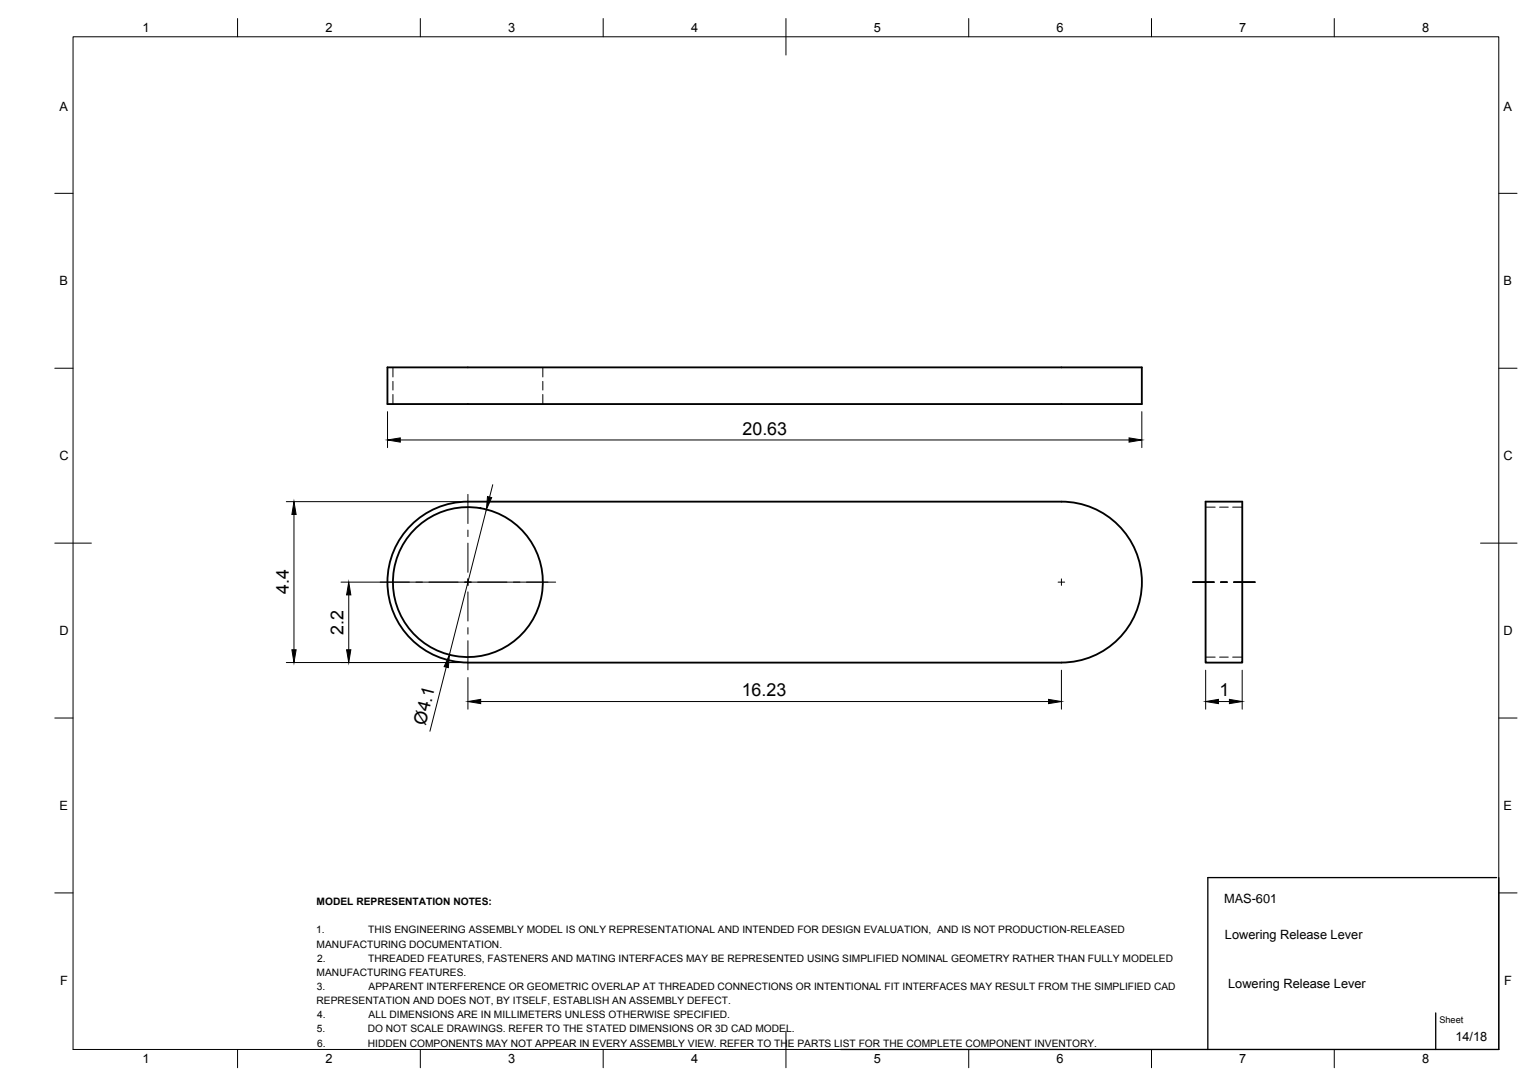
ISO-10303-21;
HEADER;
FILE_DESCRIPTION((''),'2;1');
FILE_NAME('Lowering Release Lever.step','2026-10-06T07:37:42+05:00',(''),(''),'','','');
FILE_SCHEMA (('AUTOMOTIVE_DESIGN { 1 0 10303 214 3 1 1 }'));
ENDSEC;
DATA;
#10=MECHANICAL_DESIGN_GEOMETRIC_PRESENTATION_REPRESENTATION('',(#382),#18757);
#348=SHAPE_REPRESENTATION_RELATIONSHIP('SRR','None',#18866,#365) ;
#365=ADVANCED_BREP_SHAPE_REPRESENTATION('',(#399),#18749) ;
#382=STYLED_ITEM('',(#18960),#399) ;
#399=MANIFOLD_SOLID_BREP('Lowering Release Lever',#9551) ;
#585=CYLINDRICAL_SURFACE('',#10206,2.05) ;
#586=CYLINDRICAL_SURFACE('',#10210,2.2) ;
#587=CYLINDRICAL_SURFACE('',#10214,2.20000000000001) ;
#727=FACE_BOUND('',#1939,.T.) ;
#728=FACE_BOUND('',#1941,.T.) ;
#902=PLANE('',#10209) ;
#903=PLANE('',#10213) ;
#904=PLANE('',#10217) ;
#905=PLANE('',#10218) ;
#1338=FACE_OUTER_BOUND('',#1933,.T.) ;
#1339=FACE_OUTER_BOUND('',#1934,.T.) ;
#1340=FACE_OUTER_BOUND('',#1935,.T.) ;
#1341=FACE_OUTER_BOUND('',#1936,.T.) ;
#1342=FACE_OUTER_BOUND('',#1937,.T.) ;
#1343=FACE_OUTER_BOUND('',#1938,.T.) ;
#1344=FACE_OUTER_BOUND('',#1940,.T.) ;
#1933=EDGE_LOOP('',(#7607,#7608,#7609,#7610)) ;
#1934=EDGE_LOOP('',(#7611,#7612,#7613,#7614)) ;
#1935=EDGE_LOOP('',(#7615,#7616,#7617,#7618)) ;
#1936=EDGE_LOOP('',(#7619,#7620,#7621,#7622)) ;
#1937=EDGE_LOOP('',(#7623,#7624,#7625,#7626)) ;
#1938=EDGE_LOOP('',(#7627,#7628,#7629,#7630)) ;
#1939=EDGE_LOOP('',(#7631)) ;
#1940=EDGE_LOOP('',(#7632,#7633,#7634,#7635)) ;
#1941=EDGE_LOOP('',(#7636)) ;
#2637=LINE('',#15165,#3408) ;
#2638=LINE('',#15170,#3409) ;
#2639=LINE('',#15172,#3410) ;
#2640=LINE('',#15174,#3411) ;
#2641=LINE('',#15175,#3412) ;
#2642=LINE('',#15181,#3413) ;
#2643=LINE('',#15184,#3414) ;
#2644=LINE('',#15186,#3415) ;
#2645=LINE('',#15187,#3416) ;
#3408=VECTOR('',#12041,2.05) ;
#3409=VECTOR('',#12046,10.) ;
#3410=VECTOR('',#12047,10.) ;
#3411=VECTOR('',#12048,10.) ;
#3412=VECTOR('',#12049,10.) ;
#3413=VECTOR('',#12056,10.) ;
#3414=VECTOR('',#12059,10.) ;
#3415=VECTOR('',#12060,10.) ;
#3416=VECTOR('',#12061,10.) ;
#3972=CIRCLE('',#10207,2.05) ;
#3973=CIRCLE('',#10208,2.05) ;
#3974=CIRCLE('',#10211,2.2) ;
#3975=CIRCLE('',#10212,2.2) ;
#3976=CIRCLE('',#10215,2.20000000000001) ;
#3977=CIRCLE('',#10216,2.20000000000001) ;
#4565=VERTEX_POINT('',#15162) ;
#4566=VERTEX_POINT('',#15164) ;
#4567=VERTEX_POINT('',#15168) ;
#4568=VERTEX_POINT('',#15169) ;
#4569=VERTEX_POINT('',#15171) ;
#4570=VERTEX_POINT('',#15173) ;
#4571=VERTEX_POINT('',#15177) ;
#4572=VERTEX_POINT('',#15179) ;
#4573=VERTEX_POINT('',#15183) ;
#4574=VERTEX_POINT('',#15185) ;
#5650=EDGE_CURVE('',#4565,#4565,#3972,.T.) ;
#5651=EDGE_CURVE('',#4565,#4566,#2637,.T.) ;
#5652=EDGE_CURVE('',#4566,#4566,#3973,.T.) ;
#5653=EDGE_CURVE('',#4567,#4568,#2638,.T.) ;
#5654=EDGE_CURVE('',#4568,#4569,#2639,.T.) ;
#5655=EDGE_CURVE('',#4570,#4569,#2640,.T.) ;
#5656=EDGE_CURVE('',#4567,#4570,#2641,.T.) ;
#5657=EDGE_CURVE('',#4571,#4567,#3974,.T.) ;
#5658=EDGE_CURVE('',#4572,#4570,#3975,.T.) ;
#5659=EDGE_CURVE('',#4571,#4572,#2642,.T.) ;
#5660=EDGE_CURVE('',#4573,#4571,#2643,.T.) ;
#5661=EDGE_CURVE('',#4574,#4572,#2644,.T.) ;
#5662=EDGE_CURVE('',#4573,#4574,#2645,.T.) ;
#5663=EDGE_CURVE('',#4568,#4573,#3976,.T.) ;
#5664=EDGE_CURVE('',#4569,#4574,#3977,.T.) ;
#7607=ORIENTED_EDGE('',*,*,#5650,.F.) ;
#7608=ORIENTED_EDGE('',*,*,#5651,.T.) ;
#7609=ORIENTED_EDGE('',*,*,#5652,.T.) ;
#7610=ORIENTED_EDGE('',*,*,#5651,.F.) ;
#7611=ORIENTED_EDGE('',*,*,#5653,.T.) ;
#7612=ORIENTED_EDGE('',*,*,#5654,.T.) ;
#7613=ORIENTED_EDGE('',*,*,#5655,.F.) ;
#7614=ORIENTED_EDGE('',*,*,#5656,.F.) ;
#7615=ORIENTED_EDGE('',*,*,#5657,.T.) ;
#7616=ORIENTED_EDGE('',*,*,#5656,.T.) ;
#7617=ORIENTED_EDGE('',*,*,#5658,.F.) ;
#7618=ORIENTED_EDGE('',*,*,#5659,.F.) ;
#7619=ORIENTED_EDGE('',*,*,#5660,.T.) ;
#7620=ORIENTED_EDGE('',*,*,#5659,.T.) ;
#7621=ORIENTED_EDGE('',*,*,#5661,.F.) ;
#7622=ORIENTED_EDGE('',*,*,#5662,.F.) ;
#7623=ORIENTED_EDGE('',*,*,#5663,.T.) ;
#7624=ORIENTED_EDGE('',*,*,#5662,.T.) ;
#7625=ORIENTED_EDGE('',*,*,#5664,.F.) ;
#7626=ORIENTED_EDGE('',*,*,#5654,.F.) ;
#7627=ORIENTED_EDGE('',*,*,#5664,.T.) ;
#7628=ORIENTED_EDGE('',*,*,#5661,.T.) ;
#7629=ORIENTED_EDGE('',*,*,#5658,.T.) ;
#7630=ORIENTED_EDGE('',*,*,#5655,.T.) ;
#7631=ORIENTED_EDGE('',*,*,#5650,.T.) ;
#7632=ORIENTED_EDGE('',*,*,#5663,.F.) ;
#7633=ORIENTED_EDGE('',*,*,#5653,.F.) ;
#7634=ORIENTED_EDGE('',*,*,#5657,.F.) ;
#7635=ORIENTED_EDGE('',*,*,#5660,.F.) ;
#7636=ORIENTED_EDGE('',*,*,#5652,.F.) ;
#9274=ADVANCED_FACE('',(#1338),#585,.F.) ;
#9275=ADVANCED_FACE('',(#1339),#902,.T.) ;
#9276=ADVANCED_FACE('',(#1340),#586,.T.) ;
#9277=ADVANCED_FACE('',(#1341),#903,.T.) ;
#9278=ADVANCED_FACE('',(#1342),#587,.T.) ;
#9279=ADVANCED_FACE('',(#1343,#727),#904,.T.) ;
#9280=ADVANCED_FACE('',(#1344,#728),#905,.F.) ;
#9551=CLOSED_SHELL('',(#9274,#9275,#9276,#9277,#9278,#9279,#9280)) ;
#10205=AXIS2_PLACEMENT_3D('',#15160,#12035,#12036) ;
#10206=AXIS2_PLACEMENT_3D('',#15161,#12037,#12038) ;
#10207=AXIS2_PLACEMENT_3D('',#15163,#12039,#12040) ;
#10208=AXIS2_PLACEMENT_3D('',#15166,#12042,#12043) ;
#10209=AXIS2_PLACEMENT_3D('',#15167,#12044,#12045) ;
#10210=AXIS2_PLACEMENT_3D('',#15176,#12050,#12051) ;
#10211=AXIS2_PLACEMENT_3D('',#15178,#12052,#12053) ;
#10212=AXIS2_PLACEMENT_3D('',#15180,#12054,#12055) ;
#10213=AXIS2_PLACEMENT_3D('',#15182,#12057,#12058) ;
#10214=AXIS2_PLACEMENT_3D('',#15188,#12062,#12063) ;
#10215=AXIS2_PLACEMENT_3D('',#15189,#12064,#12065) ;
#10216=AXIS2_PLACEMENT_3D('',#15190,#12066,#12067) ;
#10217=AXIS2_PLACEMENT_3D('',#15191,#12068,#12069) ;
#10218=AXIS2_PLACEMENT_3D('',#15192,#12070,#12071) ;
#12035=DIRECTION('axis',(0.,0.,1.)) ;
#12036=DIRECTION('refdir',(1.,0.,0.)) ;
#12037=DIRECTION('center_axis',(0.,1.,0.)) ;
#12038=DIRECTION('ref_axis',(1.,0.,0.)) ;
#12039=DIRECTION('center_axis',(0.,-1.,0.)) ;
#12040=DIRECTION('ref_axis',(1.,0.,0.)) ;
#12041=DIRECTION('',(0.,-1.,0.)) ;
#12042=DIRECTION('center_axis',(0.,-1.,0.)) ;
#12043=DIRECTION('ref_axis',(1.,0.,0.)) ;
#12044=DIRECTION('center_axis',(0.985548890759753,0.,-0.169391215599333)) ;
#12045=DIRECTION('ref_axis',(-0.169391215599333,0.,-0.985548890759753)) ;
#12046=DIRECTION('',(-0.169391215599333,0.,-0.985548890759753)) ;
#12047=DIRECTION('',(0.,1.,0.)) ;
#12048=DIRECTION('',(-0.169391215599333,0.,-0.985548890759753)) ;
#12049=DIRECTION('',(0.,1.,0.)) ;
#12050=DIRECTION('center_axis',(0.,1.,0.)) ;
#12051=DIRECTION('ref_axis',(-0.985548890759752,0.,0.169391215599339)) ;
#12052=DIRECTION('center_axis',(0.,1.,0.)) ;
#12053=DIRECTION('ref_axis',(-0.985548890759752,0.,0.169391215599339)) ;
#12054=DIRECTION('center_axis',(0.,1.,0.)) ;
#12055=DIRECTION('ref_axis',(-0.985548890759752,0.,0.169391215599339)) ;
#12056=DIRECTION('',(0.,1.,0.)) ;
#12057=DIRECTION('center_axis',(-0.985548890759753,0.,0.169391215599333)) ;
#12058=DIRECTION('ref_axis',(0.169391215599333,0.,0.985548890759753)) ;
#12059=DIRECTION('',(0.169391215599333,0.,0.985548890759753)) ;
#12060=DIRECTION('',(0.169391215599333,0.,0.985548890759753)) ;
#12061=DIRECTION('',(0.,1.,0.)) ;
#12062=DIRECTION('center_axis',(0.,1.,0.)) ;
#12063=DIRECTION('ref_axis',(0.985548890759754,0.,-0.16939121559933)) ;
#12064=DIRECTION('center_axis',(0.,1.,0.)) ;
#12065=DIRECTION('ref_axis',(0.985548890759754,0.,-0.16939121559933)) ;
#12066=DIRECTION('center_axis',(0.,1.,0.)) ;
#12067=DIRECTION('ref_axis',(0.985548890759754,0.,-0.16939121559933)) ;
#12068=DIRECTION('center_axis',(0.,1.,0.)) ;
#12069=DIRECTION('ref_axis',(1.,0.,0.)) ;
#12070=DIRECTION('center_axis',(0.,1.,0.)) ;
#12071=DIRECTION('ref_axis',(1.,0.,0.)) ;
#15160=CARTESIAN_POINT('',(0.,0.,0.)) ;
#15161=CARTESIAN_POINT('Origin',(90.25,47.1,160.)) ;
#15162=CARTESIAN_POINT('',(88.2,48.1,160.)) ;
#15163=CARTESIAN_POINT('Origin',(90.25,48.1,160.)) ;
#15164=CARTESIAN_POINT('',(88.2,47.1,160.)) ;
#15165=CARTESIAN_POINT('',(88.2,47.1,160.)) ;
#15166=CARTESIAN_POINT('Origin',(90.25,47.1,160.)) ;
#15167=CARTESIAN_POINT('Origin',(95.1682075596715,47.1,175.627339325681)) ;
#15168=CARTESIAN_POINT('',(95.1682075596715,47.1,175.627339325681)) ;
#15169=CARTESIAN_POINT('',(92.4182075596715,47.1,159.627339325681)) ;
#15170=CARTESIAN_POINT('',(95.1682075596715,47.1,175.627339325681)) ;
#15171=CARTESIAN_POINT('',(92.4182075596715,48.1,159.627339325681)) ;
#15172=CARTESIAN_POINT('',(92.4182075596715,47.1,159.627339325681)) ;
#15173=CARTESIAN_POINT('',(95.1682075596715,48.1,175.627339325681)) ;
#15174=CARTESIAN_POINT('',(95.1682075596715,48.1,175.627339325681)) ;
#15175=CARTESIAN_POINT('',(95.1682075596715,47.1,175.627339325681)) ;
#15176=CARTESIAN_POINT('Origin',(93.,47.1,176.)) ;
#15177=CARTESIAN_POINT('',(90.8317924403285,47.1,176.372660674319)) ;
#15178=CARTESIAN_POINT('Origin',(93.,47.1,176.)) ;
#15179=CARTESIAN_POINT('',(90.8317924403285,48.1,176.372660674319)) ;
#15180=CARTESIAN_POINT('Origin',(93.,48.1,176.)) ;
#15181=CARTESIAN_POINT('',(90.8317924403285,47.1,176.372660674319)) ;
#15182=CARTESIAN_POINT('Origin',(88.0817924403285,47.1,160.372660674319)) ;
#15183=CARTESIAN_POINT('',(88.0817924403285,47.1,160.372660674319)) ;
#15184=CARTESIAN_POINT('',(88.0817924403285,47.1,160.372660674319)) ;
#15185=CARTESIAN_POINT('',(88.0817924403285,48.1,160.372660674319)) ;
#15186=CARTESIAN_POINT('',(88.0817924403285,48.1,160.372660674319)) ;
#15187=CARTESIAN_POINT('',(88.0817924403285,47.1,160.372660674319)) ;
#15188=CARTESIAN_POINT('Origin',(90.25,47.1,160.)) ;
#15189=CARTESIAN_POINT('Origin',(90.25,47.1,160.)) ;
#15190=CARTESIAN_POINT('Origin',(90.25,48.1,160.)) ;
#15191=CARTESIAN_POINT('Origin',(91.625,48.1,168.)) ;
#15192=CARTESIAN_POINT('Origin',(91.625,47.1,168.)) ;
#18730=UNCERTAINTY_MEASURE_WITH_UNIT(LENGTH_MEASURE(0.01),#18758,
'DISTANCE_ACCURACY_VALUE',
'Maximum model space distance between geometric entities at asserted c
onnectivities') ;
#18738=UNCERTAINTY_MEASURE_WITH_UNIT(LENGTH_MEASURE(0.01),#18758,
'DISTANCE_ACCURACY_VALUE',
'Maximum model space distance between geometric entities at asserted c
onnectivities') ;
#18749=(
GEOMETRIC_REPRESENTATION_CONTEXT(3)
GLOBAL_UNCERTAINTY_ASSIGNED_CONTEXT((#18730))
GLOBAL_UNIT_ASSIGNED_CONTEXT((#18758,#18760,#18761))
REPRESENTATION_CONTEXT('','3D')
) ;
#18757=(
GEOMETRIC_REPRESENTATION_CONTEXT(3)
GLOBAL_UNCERTAINTY_ASSIGNED_CONTEXT((#18738))
GLOBAL_UNIT_ASSIGNED_CONTEXT((#18758,#18760,#18761))
REPRESENTATION_CONTEXT('','3D')
) ;
#18758=(
LENGTH_UNIT()
NAMED_UNIT(*)
SI_UNIT(.MILLI.,.METRE.)
) ;
#18760=(
NAMED_UNIT(*)
PLANE_ANGLE_UNIT()
SI_UNIT($,.RADIAN.)
) ;
#18761=(
NAMED_UNIT(*)
SI_UNIT($,.STERADIAN.)
SOLID_ANGLE_UNIT()
) ;
#18772=SHAPE_DEFINITION_REPRESENTATION(#18790,#18866) ;
#18790=PRODUCT_DEFINITION_SHAPE('',$,#18885) ;
#18866=SHAPE_REPRESENTATION('',(#10205),#18749) ;
#18874=PRODUCT_DEFINITION_CONTEXT('part definition',#18930,'design') ;
#18885=PRODUCT_DEFINITION('Lowering Release Lever',
'Lowering Release Lever',#18903,#18874) ;
#18903=PRODUCT_DEFINITION_FORMATION('',$,#18942) ;
#18930=APPLICATION_CONTEXT(
'Core Data for Automotive Mechanical Design Process') ;
#18931=PRODUCT_CONTEXT('part definition',#18930,'mechanical') ;
#18942=PRODUCT('Lowering Release Lever','Lowering Release Lever',$,(#18931)) ;
#18960=PRESENTATION_STYLE_ASSIGNMENT((#18978)) ;
#18978=SURFACE_STYLE_USAGE(.BOTH.,#18996) ;
#18996=SURFACE_SIDE_STYLE('',(#19014)) ;
#19014=SURFACE_STYLE_FILL_AREA(#19032) ;
#19032=FILL_AREA_STYLE(
'MAS-253 Metallic Sheet - Lowering Release Lever',(#19050)) ;
#19050=FILL_AREA_STYLE_COLOUR(
'MAS-253 Metallic Sheet - Lowering Release Lever',#19068) ;
#19068=COLOUR_RGB('MAS-253 Metallic Sheet - Lowering Release Lever', 0.72549020, 0.75294118, 0.79215686) ;
ENDSEC;
END-ISO-10303-21;
